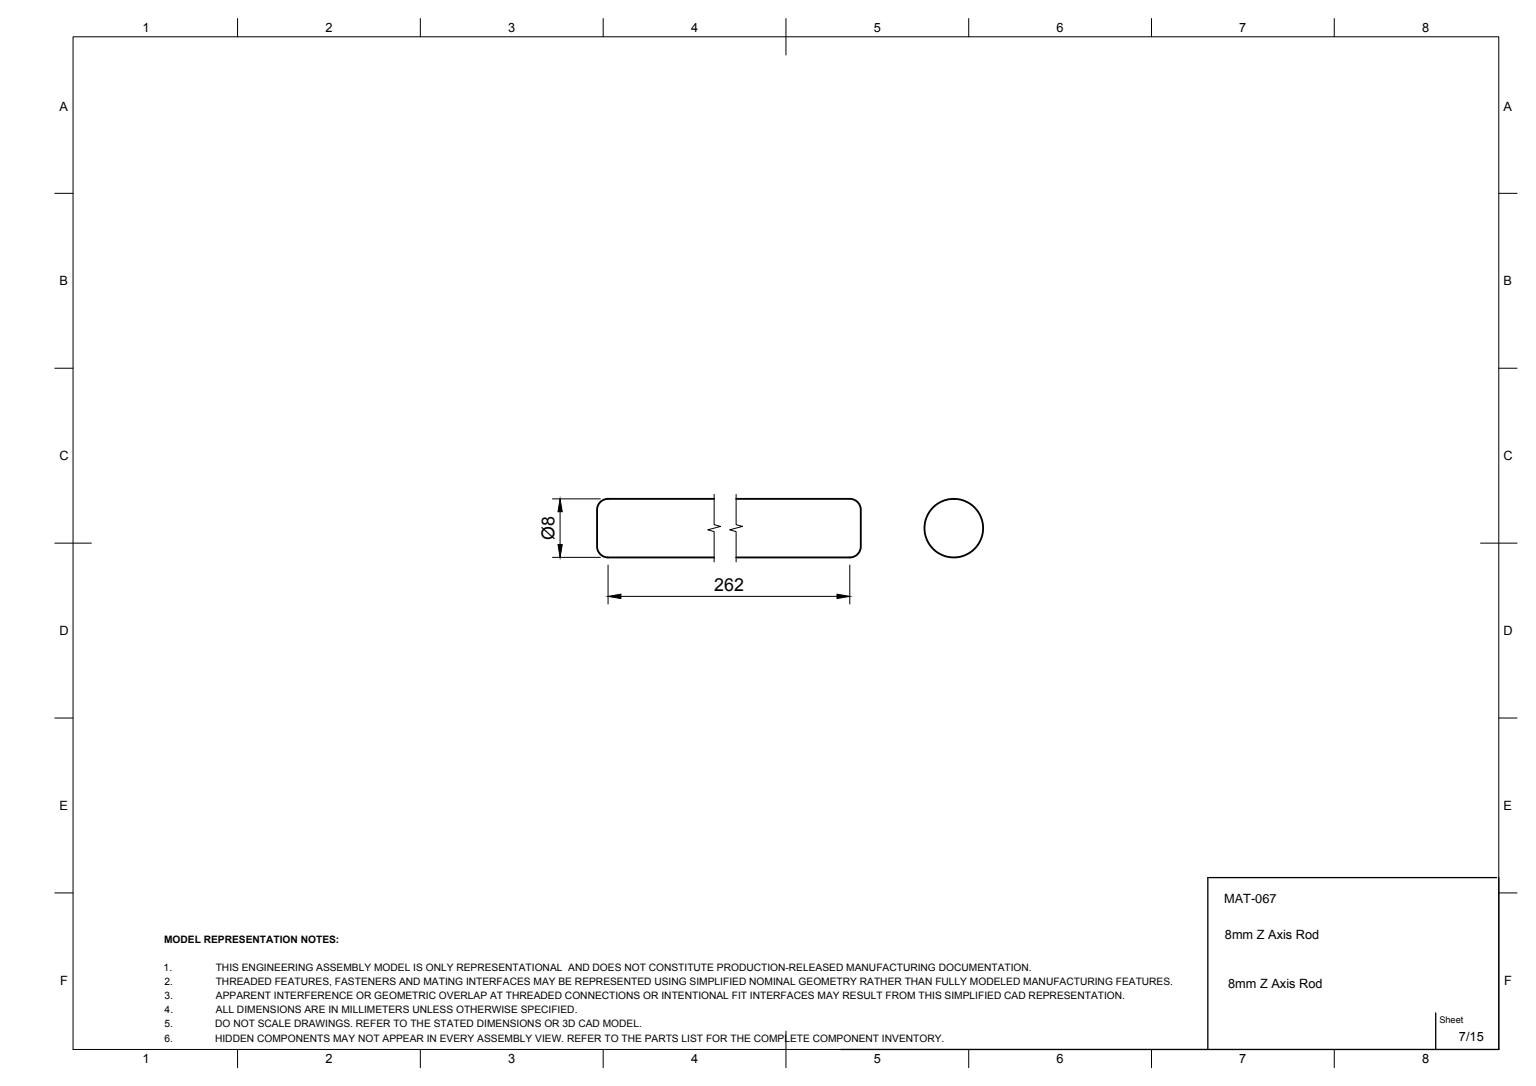
ISO-10303-21;
HEADER;
/* Generated by software containing ST-Developer
 * from STEP Tools, Inc. (www.steptools.com) 
 */

FILE_DESCRIPTION(
/* description */ ('CAx-IF Rec.Pracs.---Representation and Presentation of Product Manufa
cturing Information (PMI)---4.0---2014-10-13'),
/* implementation_level */ '2;1');

FILE_NAME(
/* name */ '8mm Z Axis Rod.step',
/* time_stamp */ '2026-10-24T16:02:03-07:00',
/* author */ (''),
/* organization */ (''),
/* preprocessor_version */ 'ST-DEVELOPER v20.2',
/* originating_system */ 'Autodesk Translation Framework v15.17.0.0',
/* authorisation */ '');

FILE_SCHEMA (('AP242_MANAGED_MODEL_BASED_3D_ENGINEERING_MIM_LF { 1 0 10303 442 2 1 4 }'));
ENDSEC;

DATA;
#10=MECHANICAL_DESIGN_GEOMETRIC_PRESENTATION_REPRESENTATION('',(#355),#6348);
#325=TOROIDAL_SURFACE('',#3789,0.0025,0.0015);
#326=TOROIDAL_SURFACE('',#3791,0.0025,0.0015);
#333=SHAPE_REPRESENTATION_RELATIONSHIP('SRR','None',#6484,#344);
#344=ADVANCED_BREP_SHAPE_REPRESENTATION('',(#366),#6332);
#355=STYLED_ITEM('',(#6605),#366);
#366=MANIFOLD_SOLID_BREP('Body1',#3394);
#445=CYLINDRICAL_SURFACE('',#3780,0.004);
#636=CIRCLE('',#3781,0.004);
#637=CIRCLE('',#3782,0.004);
#638=CIRCLE('',#3783,0.004);
#639=CIRCLE('',#3784,0.004);
#640=CIRCLE('',#3786,0.0025);
#641=CIRCLE('',#3788,0.0025);
#642=CIRCLE('',#3790,0.0015);
#643=CIRCLE('',#3792,0.0015);
#814=FACE_OUTER_BOUND('',#1009,.T.);
#815=FACE_OUTER_BOUND('',#1010,.T.);
#816=FACE_OUTER_BOUND('',#1011,.T.);
#817=FACE_OUTER_BOUND('',#1012,.T.);
#818=FACE_OUTER_BOUND('',#1013,.T.);
#1009=EDGE_LOOP('',(#2963,#2964,#2965,#2966,#2967,#2968));
#1010=EDGE_LOOP('',(#2969));
#1011=EDGE_LOOP('',(#2970));
#1012=EDGE_LOOP('',(#2971,#2972,#2973,#2974,#2975));
#1013=EDGE_LOOP('',(#2976,#2977,#2978,#2979,#2980));
#1282=LINE('',#6019,#1515);
#1515=VECTOR('',#4706,0.004);
#1776=VERTEX_POINT('',#6015);
#1777=VERTEX_POINT('',#6016);
#1778=VERTEX_POINT('',#6018);
#1779=VERTEX_POINT('',#6020);
#1780=VERTEX_POINT('',#6025);
#1781=VERTEX_POINT('',#6028);
#2180=EDGE_CURVE('',#1776,#1777,#636,.T.);
#2181=EDGE_CURVE('',#1777,#1778,#1282,.T.);
#2182=EDGE_CURVE('',#1778,#1779,#637,.F.);
#2183=EDGE_CURVE('',#1779,#1778,#638,.F.);
#2184=EDGE_CURVE('',#1777,#1776,#639,.T.);
#2185=EDGE_CURVE('',#1780,#1780,#640,.T.);
#2186=EDGE_CURVE('',#1781,#1781,#641,.F.);
#2187=EDGE_CURVE('',#1776,#1781,#642,.T.);
#2188=EDGE_CURVE('',#1780,#1779,#643,.T.);
#2963=ORIENTED_EDGE('',*,*,#2180,.T.);
#2964=ORIENTED_EDGE('',*,*,#2181,.T.);
#2965=ORIENTED_EDGE('',*,*,#2182,.T.);
#2966=ORIENTED_EDGE('',*,*,#2183,.T.);
#2967=ORIENTED_EDGE('',*,*,#2181,.F.);
#2968=ORIENTED_EDGE('',*,*,#2184,.T.);
#2969=ORIENTED_EDGE('',*,*,#2185,.T.);
#2970=ORIENTED_EDGE('',*,*,#2186,.T.);
#2971=ORIENTED_EDGE('',*,*,#2180,.F.);
#2972=ORIENTED_EDGE('',*,*,#2187,.T.);
#2973=ORIENTED_EDGE('',*,*,#2186,.F.);
#2974=ORIENTED_EDGE('',*,*,#2187,.F.);
#2975=ORIENTED_EDGE('',*,*,#2184,.F.);
#2976=ORIENTED_EDGE('',*,*,#2185,.F.);
#2977=ORIENTED_EDGE('',*,*,#2188,.T.);
#2978=ORIENTED_EDGE('',*,*,#2182,.F.);
#2979=ORIENTED_EDGE('',*,*,#2183,.F.);
#2980=ORIENTED_EDGE('',*,*,#2188,.F.);
#3197=PLANE('',#3785);
#3198=PLANE('',#3787);
#3337=ADVANCED_FACE('',(#814),#445,.T.);
#3338=ADVANCED_FACE('',(#815),#3197,.T.);
#3339=ADVANCED_FACE('',(#816),#3198,.F.);
#3340=ADVANCED_FACE('',(#817),#325,.T.);
#3341=ADVANCED_FACE('',(#818),#326,.T.);
#3394=CLOSED_SHELL('',(#3337,#3338,#3339,#3340,#3341));
#3779=AXIS2_PLACEMENT_3D('',#6013,#4700,#4701);
#3780=AXIS2_PLACEMENT_3D('',#6014,#4702,#4703);
#3781=AXIS2_PLACEMENT_3D('',#6017,#4704,#4705);
#3782=AXIS2_PLACEMENT_3D('',#6021,#4707,#4708);
#3783=AXIS2_PLACEMENT_3D('',#6022,#4709,#4710);
#3784=AXIS2_PLACEMENT_3D('',#6023,#4711,#4712);
#3785=AXIS2_PLACEMENT_3D('',#6024,#4713,#4714);
#3786=AXIS2_PLACEMENT_3D('',#6026,#4715,#4716);
#3787=AXIS2_PLACEMENT_3D('',#6027,#4717,#4718);
#3788=AXIS2_PLACEMENT_3D('',#6029,#4719,#4720);
#3789=AXIS2_PLACEMENT_3D('',#6030,#4721,#4722);
#3790=AXIS2_PLACEMENT_3D('',#6031,#4723,#4724);
#3791=AXIS2_PLACEMENT_3D('',#6032,#4725,#4726);
#3792=AXIS2_PLACEMENT_3D('',#6033,#4727,#4728);
#4700=DIRECTION('axis',(0.,0.,1.));
#4701=DIRECTION('refdir',(1.,0.,0.));
#4702=DIRECTION('center_axis',(0.,0.,-1.));
#4703=DIRECTION('ref_axis',(-1.,0.,0.));
#4704=DIRECTION('center_axis',(0.,0.,1.));
#4705=DIRECTION('ref_axis',(1.,0.,0.));
#4706=DIRECTION('',(0.,0.,1.));
#4707=DIRECTION('center_axis',(0.,0.,1.));
#4708=DIRECTION('ref_axis',(1.,0.,0.));
#4709=DIRECTION('center_axis',(0.,0.,1.));
#4710=DIRECTION('ref_axis',(1.,0.,0.));
#4711=DIRECTION('center_axis',(0.,0.,1.));
#4712=DIRECTION('ref_axis',(1.,0.,0.));
#4713=DIRECTION('center_axis',(0.,0.,1.));
#4714=DIRECTION('ref_axis',(1.,0.,0.));
#4715=DIRECTION('center_axis',(0.,0.,1.));
#4716=DIRECTION('ref_axis',(1.,0.,0.));
#4717=DIRECTION('center_axis',(0.,0.,1.));
#4718=DIRECTION('ref_axis',(1.,0.,0.));
#4719=DIRECTION('center_axis',(0.,0.,1.));
#4720=DIRECTION('ref_axis',(1.,0.,0.));
#4721=DIRECTION('center_axis',(0.,0.,1.));
#4722=DIRECTION('ref_axis',(1.,0.,0.));
#4723=DIRECTION('center_axis',(1.22464679914735E-16,-1.,0.));
#4724=DIRECTION('ref_axis',(-1.,-1.22464679914735E-16,0.));
#4725=DIRECTION('center_axis',(0.,0.,1.));
#4726=DIRECTION('ref_axis',(1.,0.,0.));
#4727=DIRECTION('center_axis',(1.22464679914735E-16,-1.,0.));
#4728=DIRECTION('ref_axis',(-1.,-1.22464679914735E-16,0.));
#6013=CARTESIAN_POINT('',(0.,0.,0.));
#6014=CARTESIAN_POINT('Origin',(0.,2.4492935982947E-19,0.265));
#6015=CARTESIAN_POINT('',(-0.004,-2.44929359829471E-19,0.0015));
#6016=CARTESIAN_POINT('',(0.004,-2.44929359829471E-19,0.00149999999999999));
#6017=CARTESIAN_POINT('Origin',(0.,2.4492935982947E-19,0.0015));
#6018=CARTESIAN_POINT('',(0.004,-2.44929359829471E-19,0.2635));
#6019=CARTESIAN_POINT('',(0.004,-2.44929359829471E-19,0.265));
#6020=CARTESIAN_POINT('',(-0.004,-2.44929359829471E-19,0.2635));
#6021=CARTESIAN_POINT('Origin',(0.,2.4492935982947E-19,0.2635));
#6022=CARTESIAN_POINT('Origin',(0.,2.4492935982947E-19,0.2635));
#6023=CARTESIAN_POINT('Origin',(0.,2.4492935982947E-19,0.0015));
#6024=CARTESIAN_POINT('Origin',(0.,0.,0.265));
#6025=CARTESIAN_POINT('',(-0.0025,-6.12323399573683E-20,0.265));
#6026=CARTESIAN_POINT('Origin',(0.,2.4492935982947E-19,0.265));
#6027=CARTESIAN_POINT('Origin',(0.,0.,0.));
#6028=CARTESIAN_POINT('',(-0.0025,-6.12323399573683E-20,0.));
#6029=CARTESIAN_POINT('Origin',(0.,2.4492935982947E-19,0.));
#6030=CARTESIAN_POINT('Origin',(0.,2.4492935982947E-19,0.0015));
#6031=CARTESIAN_POINT('Origin',(-0.0025,-6.12323399573683E-20,0.0015));
#6032=CARTESIAN_POINT('Origin',(0.,2.4492935982947E-19,0.2635));
#6033=CARTESIAN_POINT('Origin',(-0.0025,-6.12323399573683E-20,0.2635));
#6307=UNCERTAINTY_MEASURE_WITH_UNIT(LENGTH_MEASURE(1.E-5),#6349,
'DISTANCE_ACCURACY_VALUE',
'Maximum model space distance between geometric entities at asserted c
onnectivities');
#6323=UNCERTAINTY_MEASURE_WITH_UNIT(LENGTH_MEASURE(1.E-5),#6349,
'DISTANCE_ACCURACY_VALUE',
'Maximum model space distance between geometric entities at asserted c
onnectivities');
#6332=(
GEOMETRIC_REPRESENTATION_CONTEXT(3)
GLOBAL_UNCERTAINTY_ASSIGNED_CONTEXT((#6307))
GLOBAL_UNIT_ASSIGNED_CONTEXT((#6349,#6350,#6351))
REPRESENTATION_CONTEXT('','3D')
);
#6348=(
GEOMETRIC_REPRESENTATION_CONTEXT(3)
GLOBAL_UNCERTAINTY_ASSIGNED_CONTEXT((#6323))
GLOBAL_UNIT_ASSIGNED_CONTEXT((#6349,#6350,#6351))
REPRESENTATION_CONTEXT('','3D')
);
#6349=(
LENGTH_UNIT()
NAMED_UNIT(*)
SI_UNIT($,.METRE.)
);
#6350=(
NAMED_UNIT(*)
PLANE_ANGLE_UNIT()
SI_UNIT($,.RADIAN.)
);
#6351=(
NAMED_UNIT(*)
SI_UNIT($,.STERADIAN.)
SOLID_ANGLE_UNIT()
);
#6360=SHAPE_DEFINITION_REPRESENTATION(#6384,#6484);
#6384=PRODUCT_DEFINITION_SHAPE('',$,#6509);
#6484=SHAPE_REPRESENTATION('',(#3779),#6332);
#6500=PRODUCT_DEFINITION_CONTEXT('part definition',#6574,'design');
#6509=PRODUCT_DEFINITION('8mm Z Axis Rod','8mm Z Axis Rod',#6533,#6500);
#6533=PRODUCT_DEFINITION_FORMATION('',$,#6584);
#6574=APPLICATION_CONTEXT('Managed model based 3d engineering');
#6575=PRODUCT_CONTEXT('part definition',#6574,'mechanical');
#6584=PRODUCT('8mm Z Axis Rod','8mm Z Axis Rod',
'LEGAL AND USAGE DISCLAIMER: this Data/Model is provided \X2\201C\X0\A
S IS\X2\201D\X0\ for informational and representational only. It is a 
geometric approximation and is NOT engineered, certified, or guarantee
d for dimensional accuracy, exact tolerances, or production-level prec
ision. Vendor disclaims all implied warranties including fitness for a
 particular purpose. DO NOT USE FOR DIRECT PHYSICAL MANUFACTURING, AUT
OMATED PRODUCTION, OR SAFETY-CRITICAL SYSTEMS without independent engi
neering verification and resolution of any design discrepancies.',(#6575));
#6605=PRESENTATION_STYLE_ASSIGNMENT((#6611));
#6611=SURFACE_STYLE_USAGE(.BOTH.,#6617);
#6617=SURFACE_SIDE_STYLE('',(#6623));
#6623=SURFACE_STYLE_FILL_AREA(#6629);
#6629=FILL_AREA_STYLE('Opaque(48,59,150)',(#6635));
#6635=FILL_AREA_STYLE_COLOUR('Opaque(48,59,150)',#6641);
#6641=COLOUR_RGB('Opaque(48,59,150)',0.188235294117647,0.231372549019608,
0.588235294117647);
ENDSEC;
END-ISO-10303-21;
